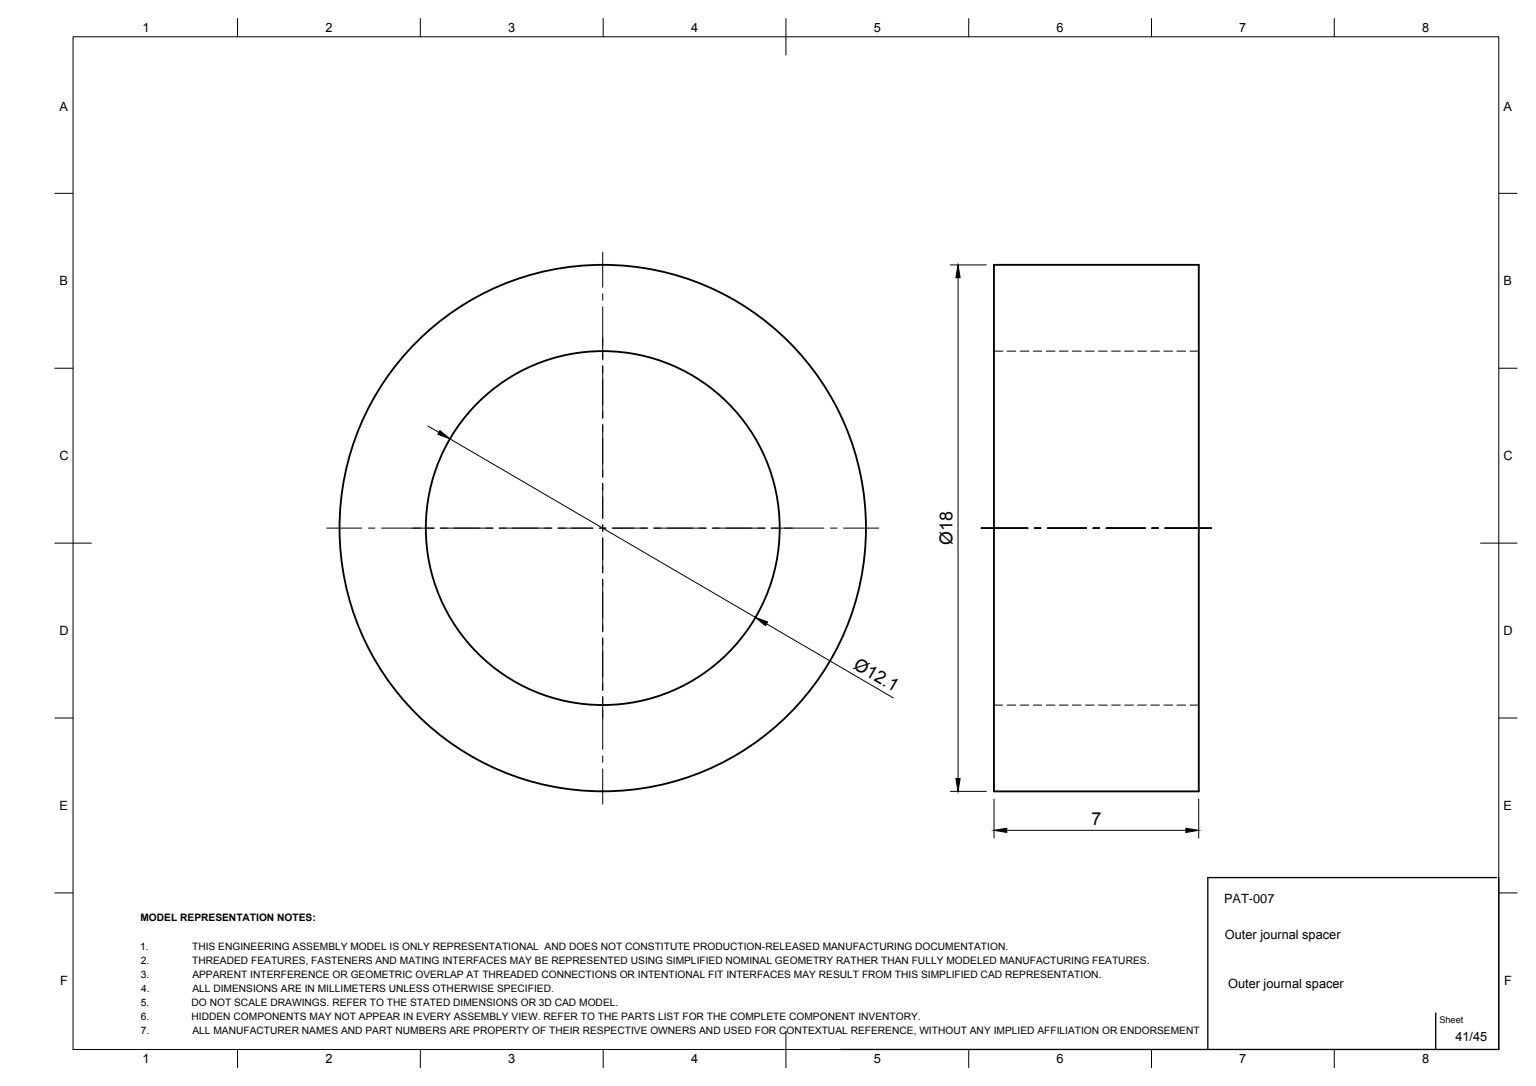
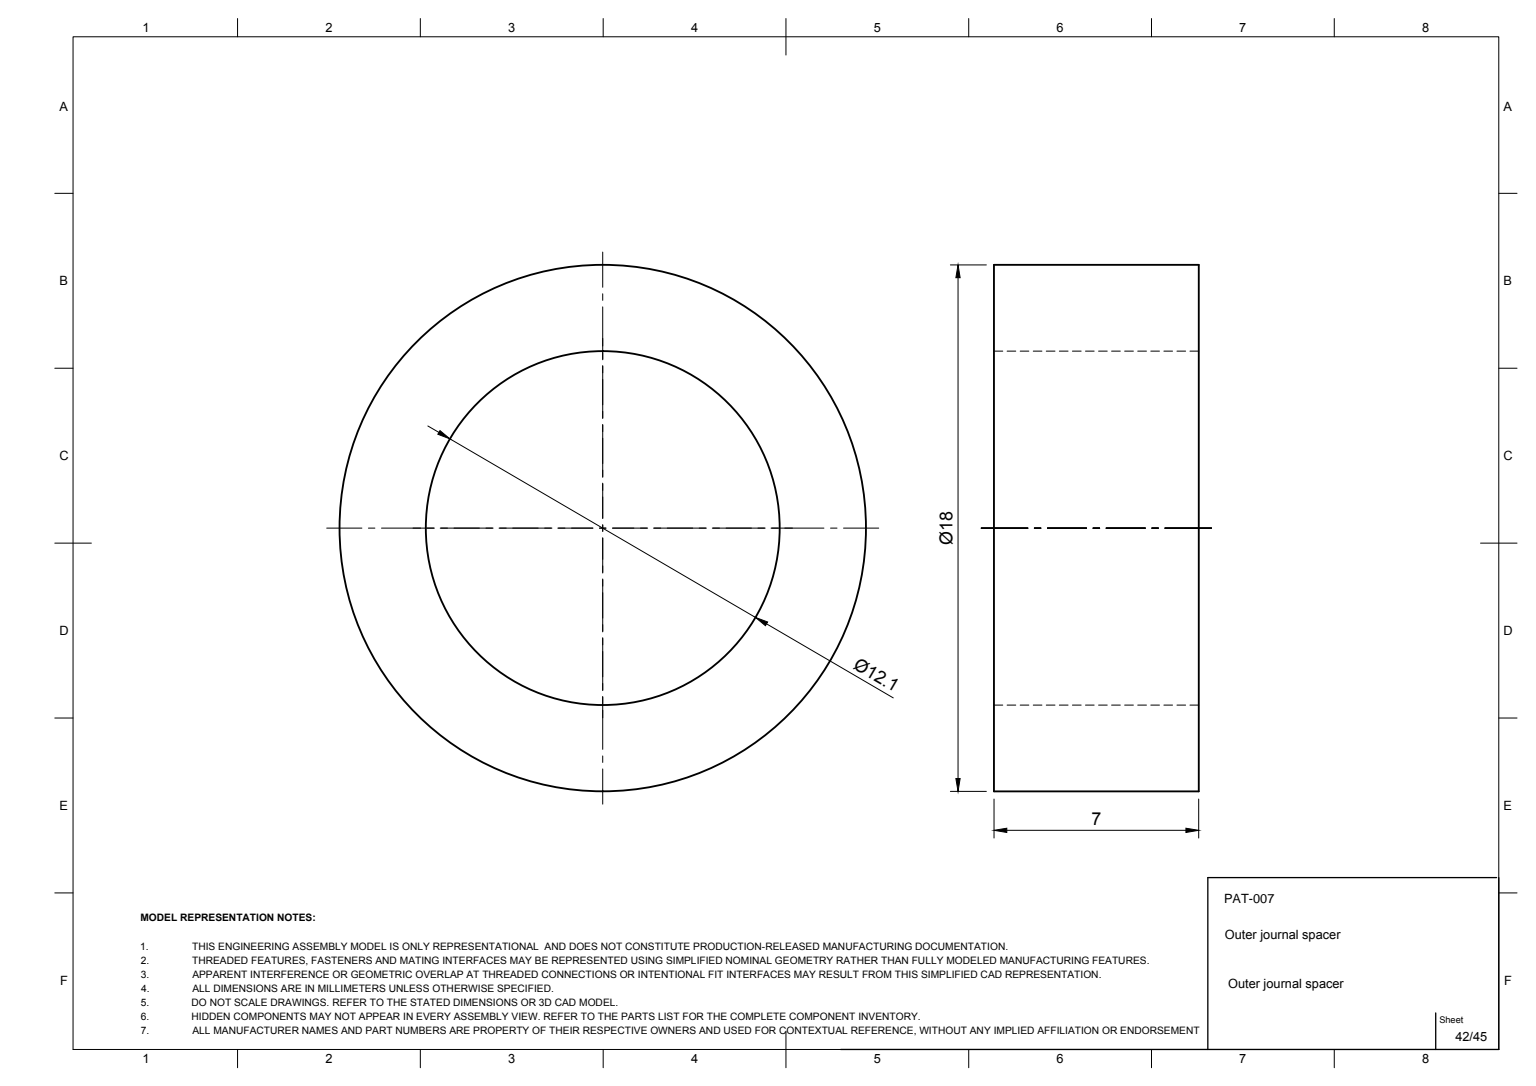
ISO-10303-21;
HEADER;
/* Generated by software containing ST-Developer
 * from STEP Tools, Inc. (www.steptools.com) 
 */

FILE_DESCRIPTION(
/* description */ ('Bearing friction torque test rig'),
/* implementation_level */ '2;1');

FILE_NAME(
/* name */ 'Outer journal spacer.step',
/* time_stamp */ '2026-10-28T03:24:04-07:00',
/* author */ (''),
/* organization */ (''),
/* preprocessor_version */ 'ST-DEVELOPER v20.2',
/* originating_system */ 'Autodesk Translation Framework v15.17.0.0',
/* authorisation */ '');

FILE_SCHEMA (('AUTOMOTIVE_DESIGN { 1 0 10303 214 3 1 1 }'));
ENDSEC;

DATA;
#10=MECHANICAL_DESIGN_GEOMETRIC_PRESENTATION_REPRESENTATION('',(#587),#14822);
#494=SHAPE_REPRESENTATION_RELATIONSHIP('SRR','None',#15036,#533);
#533=ADVANCED_BREP_SHAPE_REPRESENTATION('',(#638),#14816);
#587=STYLED_ITEM('',(#15277),#638);
#638=MANIFOLD_SOLID_BREP('Body1',#7706);
#848=FACE_BOUND('',#2149,.T.);
#849=FACE_BOUND('',#2151,.T.);
#1073=PLANE('',#9060);
#1074=PLANE('',#9061);
#1497=FACE_OUTER_BOUND('',#2146,.T.);
#1498=FACE_OUTER_BOUND('',#2147,.T.);
#1499=FACE_OUTER_BOUND('',#2148,.T.);
#1500=FACE_OUTER_BOUND('',#2150,.T.);
#2146=EDGE_LOOP('',(#6844,#6845,#6846,#6847));
#2147=EDGE_LOOP('',(#6848,#6849,#6850,#6851));
#2148=EDGE_LOOP('',(#6852));
#2149=EDGE_LOOP('',(#6853));
#2150=EDGE_LOOP('',(#6854));
#2151=EDGE_LOOP('',(#6855));
#2618=LINE('',#14329,#3062);
#2619=LINE('',#14335,#3063);
#3062=VECTOR('',#11393,0.605);
#3063=VECTOR('',#11400,0.9);
#3510=CIRCLE('',#9055,0.605);
#3511=CIRCLE('',#9056,0.605);
#3512=CIRCLE('',#9058,0.9);
#3513=CIRCLE('',#9059,0.9);
#4133=VERTEX_POINT('',#14326);
#4134=VERTEX_POINT('',#14328);
#4135=VERTEX_POINT('',#14332);
#4136=VERTEX_POINT('',#14334);
#5048=EDGE_CURVE('',#4133,#4133,#3510,.T.);
#5049=EDGE_CURVE('',#4133,#4134,#2618,.T.);
#5050=EDGE_CURVE('',#4134,#4134,#3511,.T.);
#5051=EDGE_CURVE('',#4135,#4135,#3512,.T.);
#5052=EDGE_CURVE('',#4135,#4136,#2619,.T.);
#5053=EDGE_CURVE('',#4136,#4136,#3513,.T.);
#6844=ORIENTED_EDGE('',*,*,#5048,.F.);
#6845=ORIENTED_EDGE('',*,*,#5049,.T.);
#6846=ORIENTED_EDGE('',*,*,#5050,.T.);
#6847=ORIENTED_EDGE('',*,*,#5049,.F.);
#6848=ORIENTED_EDGE('',*,*,#5051,.F.);
#6849=ORIENTED_EDGE('',*,*,#5052,.T.);
#6850=ORIENTED_EDGE('',*,*,#5053,.T.);
#6851=ORIENTED_EDGE('',*,*,#5052,.F.);
#6852=ORIENTED_EDGE('',*,*,#5051,.T.);
#6853=ORIENTED_EDGE('',*,*,#5048,.T.);
#6854=ORIENTED_EDGE('',*,*,#5053,.F.);
#6855=ORIENTED_EDGE('',*,*,#5050,.F.);
#7191=CYLINDRICAL_SURFACE('',#9054,0.605);
#7192=CYLINDRICAL_SURFACE('',#9057,0.9);
#7608=ADVANCED_FACE('',(#1497),#7191,.F.);
#7609=ADVANCED_FACE('',(#1498),#7192,.T.);
#7610=ADVANCED_FACE('',(#1499,#848),#1073,.T.);
#7611=ADVANCED_FACE('',(#1500,#849),#1074,.F.);
#7706=CLOSED_SHELL('',(#7608,#7609,#7610,#7611));
#9053=AXIS2_PLACEMENT_3D('',#14324,#11387,#11388);
#9054=AXIS2_PLACEMENT_3D('',#14325,#11389,#11390);
#9055=AXIS2_PLACEMENT_3D('',#14327,#11391,#11392);
#9056=AXIS2_PLACEMENT_3D('',#14330,#11394,#11395);
#9057=AXIS2_PLACEMENT_3D('',#14331,#11396,#11397);
#9058=AXIS2_PLACEMENT_3D('',#14333,#11398,#11399);
#9059=AXIS2_PLACEMENT_3D('',#14336,#11401,#11402);
#9060=AXIS2_PLACEMENT_3D('',#14337,#11403,#11404);
#9061=AXIS2_PLACEMENT_3D('',#14338,#11405,#11406);
#11387=DIRECTION('axis',(0.,0.,1.));
#11388=DIRECTION('refdir',(1.,0.,0.));
#11389=DIRECTION('center_axis',(0.,1.,0.));
#11390=DIRECTION('ref_axis',(1.,0.,0.));
#11391=DIRECTION('center_axis',(0.,-1.,0.));
#11392=DIRECTION('ref_axis',(1.,0.,0.));
#11393=DIRECTION('',(0.,-1.,0.));
#11394=DIRECTION('center_axis',(0.,-1.,0.));
#11395=DIRECTION('ref_axis',(1.,0.,0.));
#11396=DIRECTION('center_axis',(0.,1.,0.));
#11397=DIRECTION('ref_axis',(1.,0.,0.));
#11398=DIRECTION('center_axis',(0.,1.,0.));
#11399=DIRECTION('ref_axis',(1.,0.,0.));
#11400=DIRECTION('',(0.,-1.,0.));
#11401=DIRECTION('center_axis',(0.,1.,0.));
#11402=DIRECTION('ref_axis',(1.,0.,0.));
#11403=DIRECTION('center_axis',(0.,1.,0.));
#11404=DIRECTION('ref_axis',(1.,0.,0.));
#11405=DIRECTION('center_axis',(0.,1.,0.));
#11406=DIRECTION('ref_axis',(1.,0.,0.));
#14324=CARTESIAN_POINT('',(0.,0.,0.));
#14325=CARTESIAN_POINT('Origin',(0.,-8.2,7.));
#14326=CARTESIAN_POINT('',(-0.605,-7.5,7.));
#14327=CARTESIAN_POINT('Origin',(0.,-7.5,7.));
#14328=CARTESIAN_POINT('',(-0.605,-8.2,7.));
#14329=CARTESIAN_POINT('',(-0.605,-8.2,7.));
#14330=CARTESIAN_POINT('Origin',(0.,-8.2,7.));
#14331=CARTESIAN_POINT('Origin',(0.,-8.2,7.));
#14332=CARTESIAN_POINT('',(-0.9,-7.5,7.));
#14333=CARTESIAN_POINT('Origin',(0.,-7.5,7.));
#14334=CARTESIAN_POINT('',(-0.9,-8.2,7.));
#14335=CARTESIAN_POINT('',(-0.9,-8.2,7.));
#14336=CARTESIAN_POINT('Origin',(0.,-8.2,7.));
#14337=CARTESIAN_POINT('Origin',(0.,-7.5,7.));
#14338=CARTESIAN_POINT('Origin',(0.,-8.2,7.));
#14771=UNCERTAINTY_MEASURE_WITH_UNIT(LENGTH_MEASURE(0.001),#14823,
'DISTANCE_ACCURACY_VALUE',
'Maximum model space distance between geometric entities at asserted c
onnectivities');
#14777=UNCERTAINTY_MEASURE_WITH_UNIT(LENGTH_MEASURE(0.001),#14823,
'DISTANCE_ACCURACY_VALUE',
'Maximum model space distance between geometric entities at asserted c
onnectivities');
#14816=(
GEOMETRIC_REPRESENTATION_CONTEXT(3)
GLOBAL_UNCERTAINTY_ASSIGNED_CONTEXT((#14771))
GLOBAL_UNIT_ASSIGNED_CONTEXT((#14823,#14825,#14826))
REPRESENTATION_CONTEXT('','3D')
);
#14822=(
GEOMETRIC_REPRESENTATION_CONTEXT(3)
GLOBAL_UNCERTAINTY_ASSIGNED_CONTEXT((#14777))
GLOBAL_UNIT_ASSIGNED_CONTEXT((#14823,#14825,#14826))
REPRESENTATION_CONTEXT('','3D')
);
#14823=(
LENGTH_UNIT()
NAMED_UNIT(*)
SI_UNIT(.CENTI.,.METRE.)
);
#14825=(
NAMED_UNIT(*)
PLANE_ANGLE_UNIT()
SI_UNIT($,.RADIAN.)
);
#14826=(
NAMED_UNIT(*)
SI_UNIT($,.STERADIAN.)
SOLID_ANGLE_UNIT()
);
#14865=SHAPE_DEFINITION_REPRESENTATION(#14975,#15036);
#14975=PRODUCT_DEFINITION_SHAPE('',$,#15081);
#15036=SHAPE_REPRESENTATION('',(#9053),#14816);
#15042=PRODUCT_DEFINITION_CONTEXT('part definition',#15176,'design');
#15081=PRODUCT_DEFINITION('Outer journal spacer','Outer journal spacer',
#15125,#15042);
#15125=PRODUCT_DEFINITION_FORMATION('',$,#15216);
#15176=APPLICATION_CONTEXT(
'Core Data for Automotive Mechanical Design Process');
#15177=PRODUCT_CONTEXT('part definition',#15176,'mechanical');
#15216=PRODUCT('Outer journal spacer','Outer journal spacer',
'Outer journal spacer',(#15177));
#15271=COLOUR_RGB('Sky Blue',0.24,0.69,0.87);
#15272=FILL_AREA_STYLE_COLOUR('',#15271);
#15273=FILL_AREA_STYLE('',(#15272));
#15274=SURFACE_STYLE_FILL_AREA(#15273);
#15275=SURFACE_SIDE_STYLE('',(#15274));
#15276=SURFACE_STYLE_USAGE(.BOTH.,#15275);
#15277=PRESENTATION_STYLE_ASSIGNMENT((#15276));
ENDSEC;
END-ISO-10303-21;
